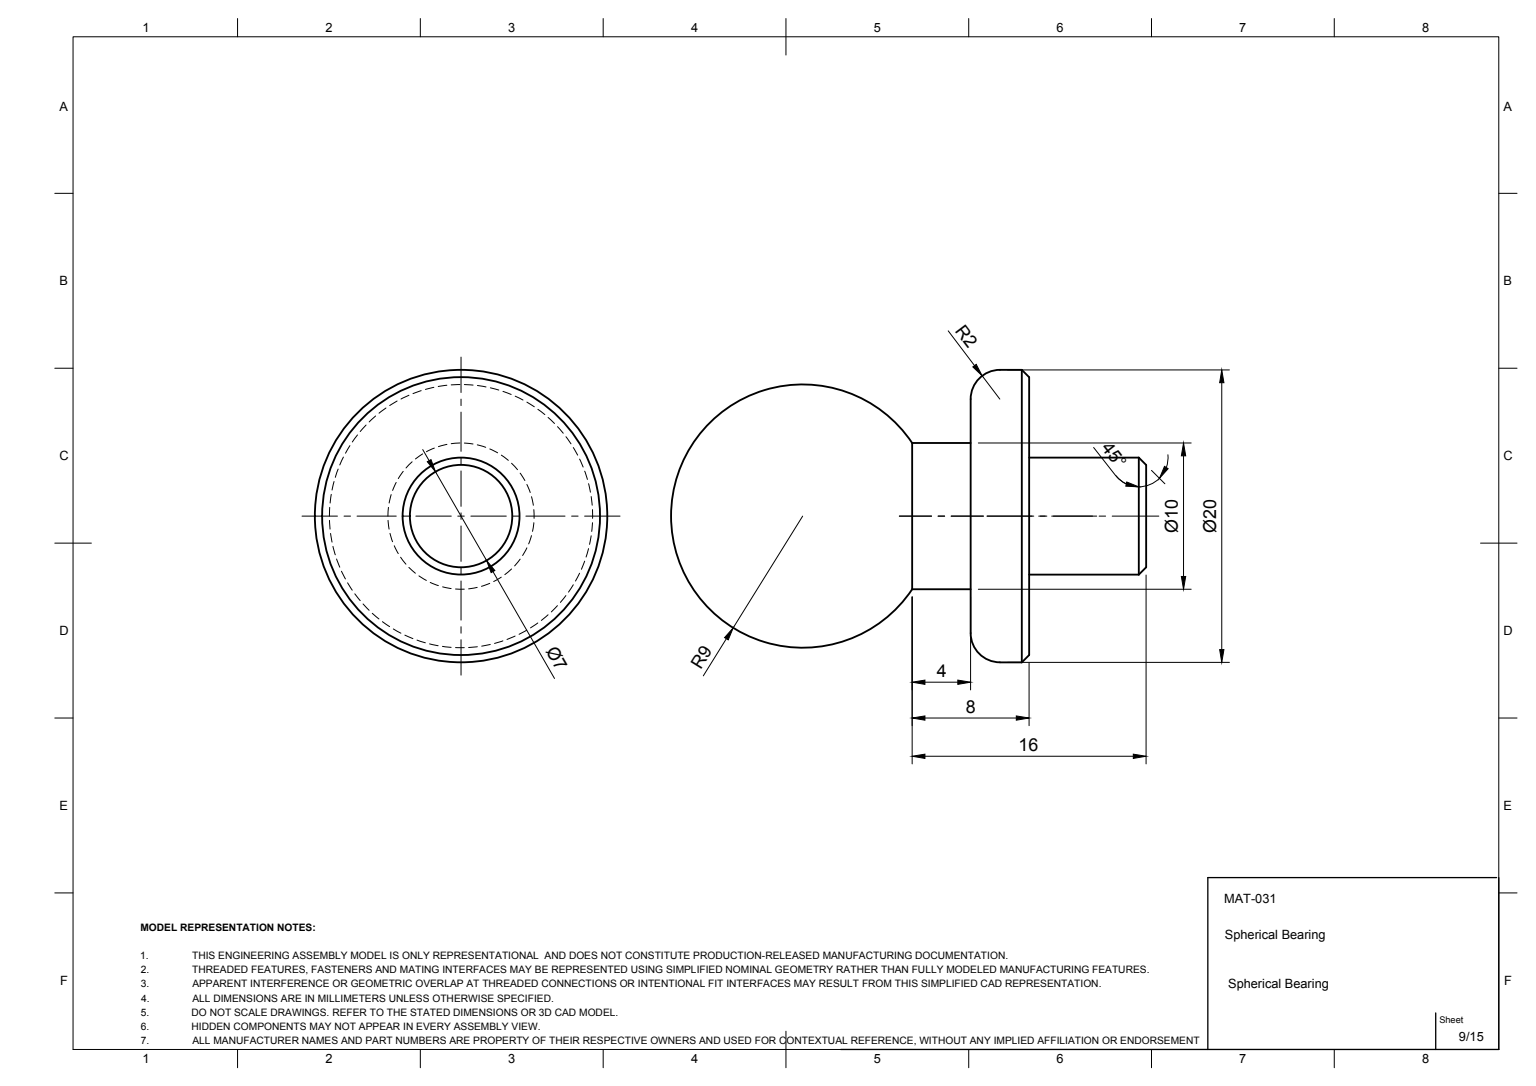
ISO-10303-21;
HEADER;
/* Generated by software containing ST-Developer
 * from STEP Tools, Inc. (www.steptools.com) 
 */

FILE_DESCRIPTION(
/* description */ ('STEP AP214'),
/* implementation_level */ '2;1');

FILE_NAME(
/* name */ 'Spherical Bearing.step',
/* time_stamp */ '2026-11-14T06:58:01-08:00',
/* author */ (''),
/* organization */ (''),
/* preprocessor_version */ 'ST-DEVELOPER v20.2',
/* originating_system */ 'Autodesk Translation Framework v15.17.0.0',
/* authorisation */ '');

FILE_SCHEMA (('AUTOMOTIVE_DESIGN { 1 0 10303 214 3 1 1 }'));
ENDSEC;

DATA;
#10=MECHANICAL_DESIGN_GEOMETRIC_PRESENTATION_REPRESENTATION('',(#1152),#38635);
#78=SPHERICAL_SURFACE('',#18050,9.);
#144=TOROIDAL_SURFACE('',#18037,8.,2.);
#872=FACE_BOUND('',#2820,.T.);
#873=FACE_BOUND('',#2823,.T.);
#874=FACE_BOUND('',#2826,.T.);
#1023=CONICAL_SURFACE('',#18043,10.,0.785398163397448);
#1024=CONICAL_SURFACE('',#18048,4.,0.78539816339745);
#1118=SHAPE_REPRESENTATION_RELATIONSHIP('SRR','None',#38691,#1132);
#1132=ADVANCED_BREP_SHAPE_REPRESENTATION('',(#1178),#38627);
#1152=STYLED_ITEM('',(#38768),#1178);
#1178=MANIFOLD_SOLID_BREP('Body1',#17618);
#1252=PLANE('',#18055);
#1253=PLANE('',#18056);
#1254=PLANE('',#18057);
#1798=FACE_OUTER_BOUND('',#2814,.T.);
#1799=FACE_OUTER_BOUND('',#2815,.T.);
#1800=FACE_OUTER_BOUND('',#2816,.T.);
#1801=FACE_OUTER_BOUND('',#2817,.T.);
#1802=FACE_OUTER_BOUND('',#2818,.T.);
#1803=FACE_OUTER_BOUND('',#2819,.T.);
#1804=FACE_OUTER_BOUND('',#2821,.T.);
#1805=FACE_OUTER_BOUND('',#2822,.T.);
#1806=FACE_OUTER_BOUND('',#2824,.T.);
#1807=FACE_OUTER_BOUND('',#2825,.T.);
#2814=EDGE_LOOP('',(#11669,#11670,#11671,#11672));
#2815=EDGE_LOOP('',(#11673,#11674,#11675,#11676));
#2816=EDGE_LOOP('',(#11677,#11678,#11679,#11680));
#2817=EDGE_LOOP('',(#11681,#11682,#11683,#11684));
#2818=EDGE_LOOP('',(#11685,#11686,#11687,#11688));
#2819=EDGE_LOOP('',(#11689,#11690));
#2820=EDGE_LOOP('',(#11691));
#2821=EDGE_LOOP('',(#11692,#11693,#11694,#11695));
#2822=EDGE_LOOP('',(#11696));
#2823=EDGE_LOOP('',(#11697));
#2824=EDGE_LOOP('',(#11698));
#2825=EDGE_LOOP('',(#11699));
#2826=EDGE_LOOP('',(#11700));
#3879=LINE('',#29949,#4823);
#3880=LINE('',#29953,#4824);
#3881=LINE('',#29959,#4825);
#3882=LINE('',#29963,#4826);
#3883=LINE('',#29973,#4827);
#4823=VECTOR('',#20434,10.);
#4824=VECTOR('',#20439,10.);
#4825=VECTOR('',#20446,4.);
#4826=VECTOR('',#20451,4.);
#4827=VECTOR('',#20462,5.);
#5675=CIRCLE('',#18038,8.);
#5676=CIRCLE('',#18039,2.);
#5677=CIRCLE('',#18040,10.);
#5678=CIRCLE('',#18042,10.);
#5679=CIRCLE('',#18044,9.5);
#5680=CIRCLE('',#18046,4.);
#5681=CIRCLE('',#18047,4.);
#5682=CIRCLE('',#18049,3.5);
#5683=CIRCLE('',#18051,9.);
#5684=CIRCLE('',#18052,5.);
#5685=CIRCLE('',#18054,5.);
#6763=VERTEX_POINT('',#29942);
#6764=VERTEX_POINT('',#29944);
#6765=VERTEX_POINT('',#29948);
#6766=VERTEX_POINT('',#29952);
#6767=VERTEX_POINT('',#29956);
#6768=VERTEX_POINT('',#29958);
#6769=VERTEX_POINT('',#29962);
#6770=VERTEX_POINT('',#29966);
#6771=VERTEX_POINT('',#29967);
#6772=VERTEX_POINT('',#29969);
#6773=VERTEX_POINT('',#29972);
#8621=EDGE_CURVE('',#6763,#6763,#5675,.T.);
#8622=EDGE_CURVE('',#6763,#6764,#5676,.T.);
#8623=EDGE_CURVE('',#6764,#6764,#5677,.T.);
#8624=EDGE_CURVE('',#6764,#6765,#3879,.T.);
#8625=EDGE_CURVE('',#6765,#6765,#5678,.T.);
#8626=EDGE_CURVE('',#6765,#6766,#3880,.T.);
#8627=EDGE_CURVE('',#6766,#6766,#5679,.T.);
#8628=EDGE_CURVE('',#6767,#6767,#5680,.T.);
#8629=EDGE_CURVE('',#6767,#6768,#3881,.T.);
#8630=EDGE_CURVE('',#6768,#6768,#5681,.T.);
#8631=EDGE_CURVE('',#6768,#6769,#3882,.T.);
#8632=EDGE_CURVE('',#6769,#6769,#5682,.T.);
#8633=EDGE_CURVE('',#6770,#6771,#5683,.T.);
#8634=EDGE_CURVE('',#6772,#6772,#5684,.T.);
#8635=EDGE_CURVE('',#6772,#6773,#3883,.T.);
#8636=EDGE_CURVE('',#6773,#6773,#5685,.T.);
#11669=ORIENTED_EDGE('',*,*,#8621,.F.);
#11670=ORIENTED_EDGE('',*,*,#8622,.T.);
#11671=ORIENTED_EDGE('',*,*,#8623,.T.);
#11672=ORIENTED_EDGE('',*,*,#8622,.F.);
#11673=ORIENTED_EDGE('',*,*,#8623,.F.);
#11674=ORIENTED_EDGE('',*,*,#8624,.T.);
#11675=ORIENTED_EDGE('',*,*,#8625,.T.);
#11676=ORIENTED_EDGE('',*,*,#8624,.F.);
#11677=ORIENTED_EDGE('',*,*,#8625,.F.);
#11678=ORIENTED_EDGE('',*,*,#8626,.T.);
#11679=ORIENTED_EDGE('',*,*,#8627,.T.);
#11680=ORIENTED_EDGE('',*,*,#8626,.F.);
#11681=ORIENTED_EDGE('',*,*,#8628,.F.);
#11682=ORIENTED_EDGE('',*,*,#8629,.T.);
#11683=ORIENTED_EDGE('',*,*,#8630,.T.);
#11684=ORIENTED_EDGE('',*,*,#8629,.F.);
#11685=ORIENTED_EDGE('',*,*,#8630,.F.);
#11686=ORIENTED_EDGE('',*,*,#8631,.T.);
#11687=ORIENTED_EDGE('',*,*,#8632,.T.);
#11688=ORIENTED_EDGE('',*,*,#8631,.F.);
#11689=ORIENTED_EDGE('',*,*,#8633,.T.);
#11690=ORIENTED_EDGE('',*,*,#8633,.F.);
#11691=ORIENTED_EDGE('',*,*,#8634,.T.);
#11692=ORIENTED_EDGE('',*,*,#8634,.F.);
#11693=ORIENTED_EDGE('',*,*,#8635,.T.);
#11694=ORIENTED_EDGE('',*,*,#8636,.T.);
#11695=ORIENTED_EDGE('',*,*,#8635,.F.);
#11696=ORIENTED_EDGE('',*,*,#8621,.T.);
#11697=ORIENTED_EDGE('',*,*,#8636,.F.);
#11698=ORIENTED_EDGE('',*,*,#8632,.F.);
#11699=ORIENTED_EDGE('',*,*,#8627,.F.);
#11700=ORIENTED_EDGE('',*,*,#8628,.T.);
#16329=CYLINDRICAL_SURFACE('',#18041,10.);
#16330=CYLINDRICAL_SURFACE('',#18045,4.);
#16331=CYLINDRICAL_SURFACE('',#18053,5.);
#16757=ADVANCED_FACE('',(#1798),#144,.T.);
#16758=ADVANCED_FACE('',(#1799),#16329,.T.);
#16759=ADVANCED_FACE('',(#1800),#1023,.T.);
#16760=ADVANCED_FACE('',(#1801),#16330,.T.);
#16761=ADVANCED_FACE('',(#1802),#1024,.T.);
#16762=ADVANCED_FACE('',(#1803,#872),#78,.T.);
#16763=ADVANCED_FACE('',(#1804),#16331,.T.);
#16764=ADVANCED_FACE('',(#1805,#873),#1252,.T.);
#16765=ADVANCED_FACE('',(#1806),#1253,.T.);
#16766=ADVANCED_FACE('',(#1807,#874),#1254,.T.);
#17618=CLOSED_SHELL('',(#16757,#16758,#16759,#16760,#16761,#16762,#16763,
#16764,#16765,#16766));
#18036=AXIS2_PLACEMENT_3D('',#29940,#20422,#20423);
#18037=AXIS2_PLACEMENT_3D('',#29941,#20424,#20425);
#18038=AXIS2_PLACEMENT_3D('',#29943,#20426,#20427);
#18039=AXIS2_PLACEMENT_3D('',#29945,#20428,#20429);
#18040=AXIS2_PLACEMENT_3D('',#29946,#20430,#20431);
#18041=AXIS2_PLACEMENT_3D('',#29947,#20432,#20433);
#18042=AXIS2_PLACEMENT_3D('',#29950,#20435,#20436);
#18043=AXIS2_PLACEMENT_3D('',#29951,#20437,#20438);
#18044=AXIS2_PLACEMENT_3D('',#29954,#20440,#20441);
#18045=AXIS2_PLACEMENT_3D('',#29955,#20442,#20443);
#18046=AXIS2_PLACEMENT_3D('',#29957,#20444,#20445);
#18047=AXIS2_PLACEMENT_3D('',#29960,#20447,#20448);
#18048=AXIS2_PLACEMENT_3D('',#29961,#20449,#20450);
#18049=AXIS2_PLACEMENT_3D('',#29964,#20452,#20453);
#18050=AXIS2_PLACEMENT_3D('',#29965,#20454,#20455);
#18051=AXIS2_PLACEMENT_3D('',#29968,#20456,#20457);
#18052=AXIS2_PLACEMENT_3D('',#29970,#20458,#20459);
#18053=AXIS2_PLACEMENT_3D('',#29971,#20460,#20461);
#18054=AXIS2_PLACEMENT_3D('',#29974,#20463,#20464);
#18055=AXIS2_PLACEMENT_3D('',#29975,#20465,#20466);
#18056=AXIS2_PLACEMENT_3D('',#29976,#20467,#20468);
#18057=AXIS2_PLACEMENT_3D('',#29977,#20469,#20470);
#20422=DIRECTION('axis',(0.,0.,1.));
#20423=DIRECTION('refdir',(1.,0.,0.));
#20424=DIRECTION('center_axis',(0.,0.,-1.));
#20425=DIRECTION('ref_axis',(-1.,0.,0.));
#20426=DIRECTION('center_axis',(0.,0.,-1.));
#20427=DIRECTION('ref_axis',(-1.,0.,0.));
#20428=DIRECTION('center_axis',(-1.22464679914735E-16,-1.,0.));
#20429=DIRECTION('ref_axis',(1.,-1.22464679914735E-16,0.));
#20430=DIRECTION('center_axis',(0.,0.,-1.));
#20431=DIRECTION('ref_axis',(-1.,0.,0.));
#20432=DIRECTION('center_axis',(0.,0.,-1.));
#20433=DIRECTION('ref_axis',(-1.,0.,0.));
#20434=DIRECTION('',(0.,0.,1.));
#20435=DIRECTION('center_axis',(0.,0.,-1.));
#20436=DIRECTION('ref_axis',(-1.,0.,0.));
#20437=DIRECTION('center_axis',(0.,0.,-1.));
#20438=DIRECTION('ref_axis',(-1.,0.,0.));
#20439=DIRECTION('',(-0.707106781186547,8.65956056235493E-17,0.707106781186548));
#20440=DIRECTION('center_axis',(0.,0.,-1.));
#20441=DIRECTION('ref_axis',(-1.,0.,0.));
#20442=DIRECTION('center_axis',(0.,0.,-1.));
#20443=DIRECTION('ref_axis',(-1.,0.,0.));
#20444=DIRECTION('center_axis',(0.,0.,-1.));
#20445=DIRECTION('ref_axis',(-1.,0.,0.));
#20446=DIRECTION('',(0.,0.,1.));
#20447=DIRECTION('center_axis',(0.,0.,-1.));
#20448=DIRECTION('ref_axis',(-1.,0.,0.));
#20449=DIRECTION('center_axis',(0.,0.,-1.));
#20450=DIRECTION('ref_axis',(-1.,0.,0.));
#20451=DIRECTION('',(-0.707106781186549,8.65956056235495E-17,0.707106781186547));
#20452=DIRECTION('center_axis',(0.,0.,-1.));
#20453=DIRECTION('ref_axis',(-1.,0.,0.));
#20454=DIRECTION('center_axis',(1.,6.12323399573677E-17,0.));
#20455=DIRECTION('ref_axis',(0.,1.,0.));
#20456=DIRECTION('center_axis',(0.,1.22464679914735E-16,-1.));
#20457=DIRECTION('ref_axis',(0.,-1.,-1.22464679914735E-16));
#20458=DIRECTION('center_axis',(0.,0.,-1.));
#20459=DIRECTION('ref_axis',(-1.,0.,0.));
#20460=DIRECTION('center_axis',(0.,0.,-1.));
#20461=DIRECTION('ref_axis',(-1.,0.,0.));
#20462=DIRECTION('',(0.,0.,1.));
#20463=DIRECTION('center_axis',(0.,0.,-1.));
#20464=DIRECTION('ref_axis',(-1.,0.,0.));
#20465=DIRECTION('center_axis',(0.,0.,-1.));
#20466=DIRECTION('ref_axis',(-1.,0.,0.));
#20467=DIRECTION('center_axis',(0.,0.,1.));
#20468=DIRECTION('ref_axis',(1.,0.,0.));
#20469=DIRECTION('center_axis',(0.,0.,1.));
#20470=DIRECTION('ref_axis',(1.,0.,0.));
#29940=CARTESIAN_POINT('',(0.,0.,0.));
#29941=CARTESIAN_POINT('Origin',(0.,0.,13.4833147735479));
#29942=CARTESIAN_POINT('',(8.,-9.79717439317882E-16,11.4833147735479));
#29943=CARTESIAN_POINT('Origin',(0.,0.,11.4833147735479));
#29944=CARTESIAN_POINT('',(10.,-1.22464679914735E-15,13.4833147735479));
#29945=CARTESIAN_POINT('Origin',(8.,-9.79717439317882E-16,13.4833147735479));
#29946=CARTESIAN_POINT('Origin',(0.,0.,13.4833147735479));
#29947=CARTESIAN_POINT('Origin',(0.,0.,0.));
#29948=CARTESIAN_POINT('',(10.,-1.22464679914735E-15,14.9833147735479));
#29949=CARTESIAN_POINT('',(10.,-1.22464679914735E-15,0.));
#29950=CARTESIAN_POINT('Origin',(0.,0.,14.9833147735479));
#29951=CARTESIAN_POINT('Origin',(0.,0.,14.9833147735479));
#29952=CARTESIAN_POINT('',(9.5,-1.16341445918999E-15,15.4833147735479));
#29953=CARTESIAN_POINT('',(10.,-1.22464679914735E-15,14.9833147735479));
#29954=CARTESIAN_POINT('Origin',(0.,0.,15.4833147735479));
#29955=CARTESIAN_POINT('Origin',(0.,0.,0.));
#29956=CARTESIAN_POINT('',(4.,-4.89858719658941E-16,15.4833147735479));
#29957=CARTESIAN_POINT('Origin',(0.,0.,15.4833147735479));
#29958=CARTESIAN_POINT('',(4.,-4.89858719658941E-16,22.9833147735479));
#29959=CARTESIAN_POINT('',(4.,-4.89858719658941E-16,0.));
#29960=CARTESIAN_POINT('Origin',(0.,0.,22.9833147735479));
#29961=CARTESIAN_POINT('Origin',(0.,0.,22.9833147735479));
#29962=CARTESIAN_POINT('',(3.5,-4.28626379701573E-16,23.4833147735479));
#29963=CARTESIAN_POINT('',(4.,-4.89858719658941E-16,22.9833147735479));
#29964=CARTESIAN_POINT('Origin',(0.,0.,23.4833147735479));
#29965=CARTESIAN_POINT('Origin',(0.,0.,0.));
#29966=CARTESIAN_POINT('',(9.,-5.51091059616309E-16,-6.74891902197836E-32));
#29967=CARTESIAN_POINT('',(-9.,-5.51091059616309E-16,-6.74891902197836E-32));
#29968=CARTESIAN_POINT('Origin',(0.,0.,0.));
#29969=CARTESIAN_POINT('',(5.,-6.12323399573676E-16,7.48331477354788));
#29970=CARTESIAN_POINT('Origin',(0.,0.,7.48331477354788));
#29971=CARTESIAN_POINT('Origin',(0.,0.,0.));
#29972=CARTESIAN_POINT('',(5.,-6.12323399573676E-16,11.4833147735479));
#29973=CARTESIAN_POINT('',(5.,-6.12323399573676E-16,0.));
#29974=CARTESIAN_POINT('Origin',(0.,0.,11.4833147735479));
#29975=CARTESIAN_POINT('Origin',(0.,5.,11.4833147735479));
#29976=CARTESIAN_POINT('Origin',(0.,3.5,23.4833147735479));
#29977=CARTESIAN_POINT('Origin',(0.,4.,15.4833147735479));
#38611=UNCERTAINTY_MEASURE_WITH_UNIT(LENGTH_MEASURE(0.01),#38636,
'DISTANCE_ACCURACY_VALUE',
'Maximum model space distance between geometric entities at asserted c
onnectivities');
#38619=UNCERTAINTY_MEASURE_WITH_UNIT(LENGTH_MEASURE(0.01),#38636,
'DISTANCE_ACCURACY_VALUE',
'Maximum model space distance between geometric entities at asserted c
onnectivities');
#38627=(
GEOMETRIC_REPRESENTATION_CONTEXT(3)
GLOBAL_UNCERTAINTY_ASSIGNED_CONTEXT((#38611))
GLOBAL_UNIT_ASSIGNED_CONTEXT((#38636,#38638,#38639))
REPRESENTATION_CONTEXT('','3D')
);
#38635=(
GEOMETRIC_REPRESENTATION_CONTEXT(3)
GLOBAL_UNCERTAINTY_ASSIGNED_CONTEXT((#38619))
GLOBAL_UNIT_ASSIGNED_CONTEXT((#38636,#38638,#38639))
REPRESENTATION_CONTEXT('','3D')
);
#38636=(
LENGTH_UNIT()
NAMED_UNIT(*)
SI_UNIT(.MILLI.,.METRE.)
);
#38638=(
NAMED_UNIT(*)
PLANE_ANGLE_UNIT()
SI_UNIT($,.RADIAN.)
);
#38639=(
NAMED_UNIT(*)
SI_UNIT($,.STERADIAN.)
SOLID_ANGLE_UNIT()
);
#38647=SHAPE_DEFINITION_REPRESENTATION(#38662,#38691);
#38662=PRODUCT_DEFINITION_SHAPE('',$,#38707);
#38691=SHAPE_REPRESENTATION('',(#18036),#38627);
#38699=PRODUCT_DEFINITION_CONTEXT('part definition',#38746,'design');
#38707=PRODUCT_DEFINITION('Spherical Bearing','Spherical Bearing',#38722,
#38699);
#38722=PRODUCT_DEFINITION_FORMATION('',$,#38755);
#38746=APPLICATION_CONTEXT(
'Core Data for Automotive Mechanical Design Process');
#38747=PRODUCT_CONTEXT('part definition',#38746,'mechanical');
#38755=PRODUCT('Spherical Bearing','Spherical Bearing',$,(#38747));
#38768=PRESENTATION_STYLE_ASSIGNMENT((#38775));
#38775=SURFACE_STYLE_USAGE(.BOTH.,#38782);
#38782=SURFACE_SIDE_STYLE('',(#38789));
#38789=SURFACE_STYLE_FILL_AREA(#38796);
#38796=FILL_AREA_STYLE('Opaque(122,133,145)',(#38803));
#38803=FILL_AREA_STYLE_COLOUR('Opaque(122,133,145)',#38810);
#38810=COLOUR_RGB('Opaque(122,133,145)',0.47843137254902,0.52156862745098,
0.568627450980392);
ENDSEC;
END-ISO-10303-21;
